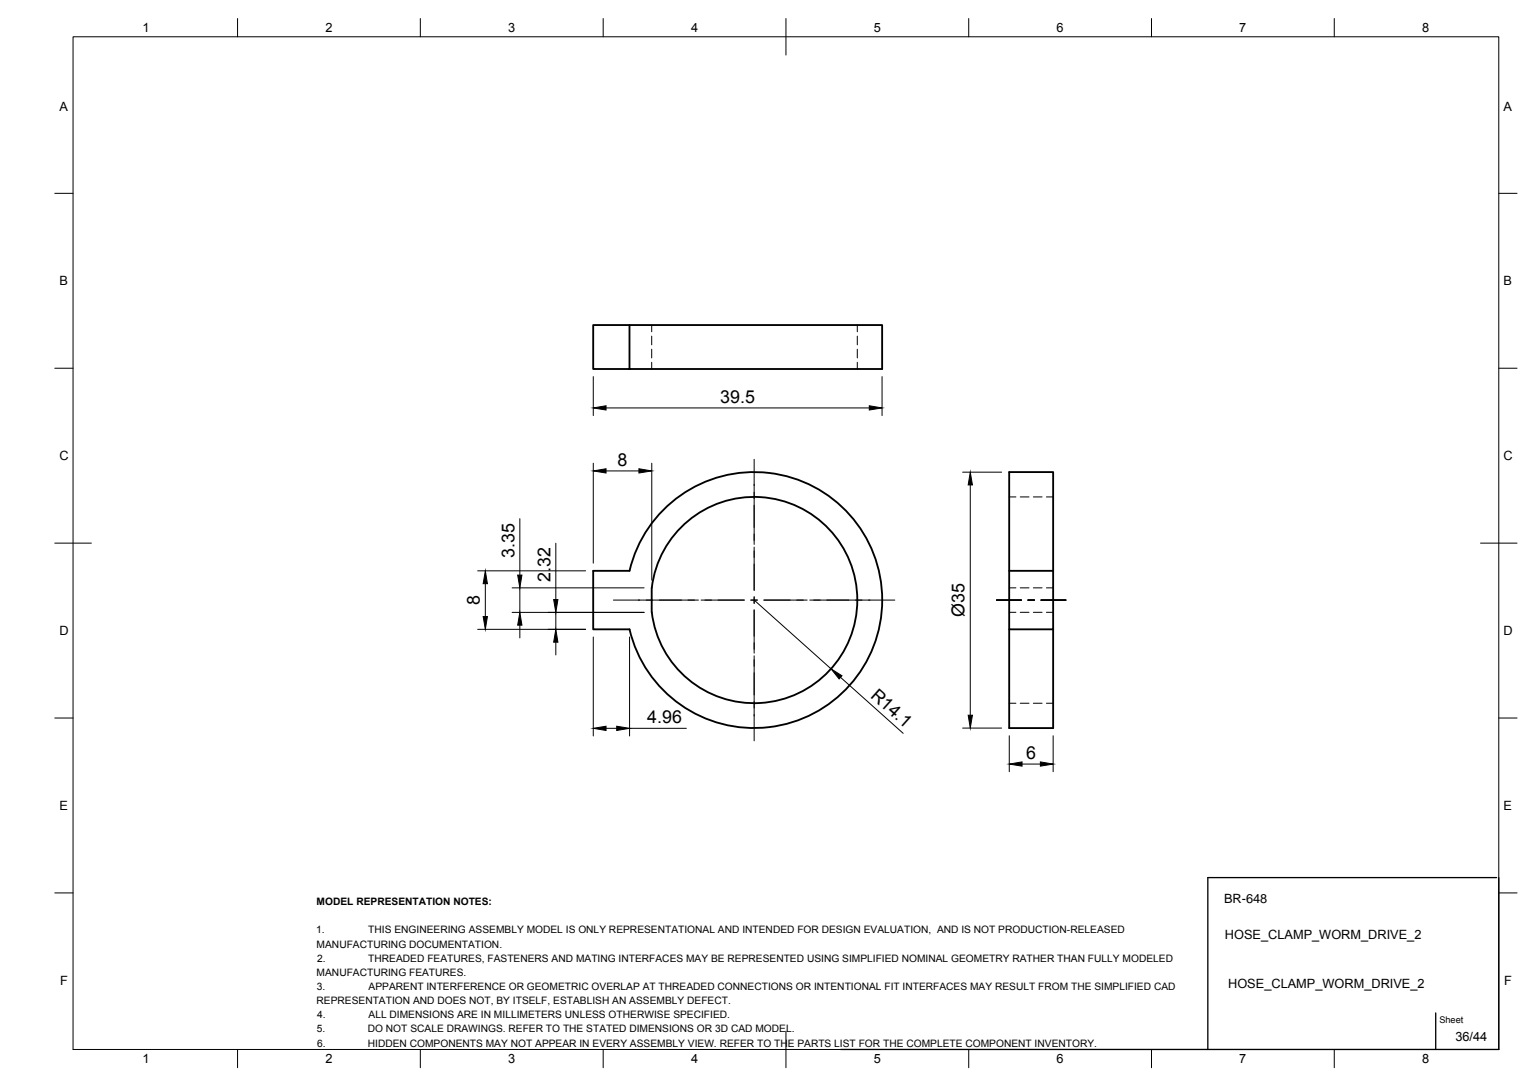
ISO-10303-21;
HEADER;
FILE_DESCRIPTION((''),'2;1');
FILE_NAME('HOSE_CLAMP_WORM_DRIVE_2.step','2026-10-01T22:05:39-07:00',(''),(''),'','','');
FILE_SCHEMA (('AUTOMOTIVE_DESIGN { 1 0 10303 214 3 1 1 }'));
ENDSEC;
DATA;
#10=MECHANICAL_DESIGN_GEOMETRIC_PRESENTATION_REPRESENTATION('',(#634),#24628);
#550=SHAPE_REPRESENTATION_RELATIONSHIP('SRR','None',#24823,#592) ;
#592=ADVANCED_BREP_SHAPE_REPRESENTATION('',(#673),#24613) ;
#634=STYLED_ITEM('',(#25034),#673) ;
#673=MANIFOLD_SOLID_BREP('HOSE_CLAMP_WORM_DRIVE_2',#13176) ;
#906=FACE_BOUND('',#4608,.T.) ;
#907=FACE_BOUND('',#4610,.T.) ;
#1693=LINE('',#23744,#2529) ;
#1694=LINE('',#23746,#2530) ;
#1695=LINE('',#23748,#2531) ;
#1696=LINE('',#23749,#2532) ;
#1697=LINE('',#23753,#2533) ;
#1698=LINE('',#23755,#2534) ;
#1699=LINE('',#23757,#2535) ;
#1700=LINE('',#23758,#2536) ;
#1701=LINE('',#23762,#2537) ;
#1702=LINE('',#23764,#2538) ;
#1703=LINE('',#23766,#2539) ;
#1704=LINE('',#23767,#2540) ;
#1705=LINE('',#23769,#2541) ;
#1706=LINE('',#23770,#2542) ;
#2529=VECTOR('',#19094,1.) ;
#2530=VECTOR('',#19095,1.) ;
#2531=VECTOR('',#19096,1.) ;
#2532=VECTOR('',#19097,1.) ;
#2533=VECTOR('',#19100,1.) ;
#2534=VECTOR('',#19101,1.) ;
#2535=VECTOR('',#19102,1.) ;
#2536=VECTOR('',#19103,1.) ;
#2537=VECTOR('',#19106,1.) ;
#2538=VECTOR('',#19107,1.) ;
#2539=VECTOR('',#19108,1.) ;
#2540=VECTOR('',#19109,1.) ;
#2541=VECTOR('',#19112,1.) ;
#2542=VECTOR('',#19113,1.) ;
#2915=CYLINDRICAL_SURFACE('',#15161,1.75) ;
#2916=CYLINDRICAL_SURFACE('',#15164,1.41) ;
#3614=FACE_OUTER_BOUND('',#4601,.T.) ;
#3615=FACE_OUTER_BOUND('',#4602,.T.) ;
#3616=FACE_OUTER_BOUND('',#4603,.T.) ;
#3617=FACE_OUTER_BOUND('',#4604,.T.) ;
#3618=FACE_OUTER_BOUND('',#4605,.T.) ;
#3619=FACE_OUTER_BOUND('',#4606,.T.) ;
#3620=FACE_OUTER_BOUND('',#4607,.T.) ;
#3621=FACE_OUTER_BOUND('',#4609,.T.) ;
#4601=EDGE_LOOP('',(#11531,#11532,#11533,#11534)) ;
#4602=EDGE_LOOP('',(#11535,#11536,#11537,#11538)) ;
#4603=EDGE_LOOP('',(#11539,#11540,#11541,#11542)) ;
#4604=EDGE_LOOP('',(#11543,#11544,#11545,#11546)) ;
#4605=EDGE_LOOP('',(#11547,#11548,#11549,#11550)) ;
#4606=EDGE_LOOP('',(#11551,#11552,#11553,#11554)) ;
#4607=EDGE_LOOP('',(#11555,#11556,#11557,#11558)) ;
#4608=EDGE_LOOP('',(#11559,#11560)) ;
#4609=EDGE_LOOP('',(#11561,#11562,#11563,#11564)) ;
#4610=EDGE_LOOP('',(#11565,#11566)) ;
#5465=CIRCLE('',#15162,1.75) ;
#5466=CIRCLE('',#15163,1.75) ;
#5467=CIRCLE('',#15165,1.41) ;
#5468=CIRCLE('',#15166,1.41) ;
#6579=VERTEX_POINT('',#23742) ;
#6580=VERTEX_POINT('',#23743) ;
#6581=VERTEX_POINT('',#23745) ;
#6582=VERTEX_POINT('',#23747) ;
#6583=VERTEX_POINT('',#23751) ;
#6584=VERTEX_POINT('',#23752) ;
#6585=VERTEX_POINT('',#23754) ;
#6586=VERTEX_POINT('',#23756) ;
#6587=VERTEX_POINT('',#23760) ;
#6588=VERTEX_POINT('',#23761) ;
#6589=VERTEX_POINT('',#23763) ;
#6590=VERTEX_POINT('',#23765) ;
#8255=EDGE_CURVE('',#6579,#6580,#1693,.T.) ;
#8256=EDGE_CURVE('',#6579,#6581,#1694,.T.) ;
#8257=EDGE_CURVE('',#6581,#6582,#1695,.T.) ;
#8258=EDGE_CURVE('',#6582,#6580,#1696,.T.) ;
#8259=EDGE_CURVE('',#6583,#6584,#1697,.T.) ;
#8260=EDGE_CURVE('',#6585,#6583,#1698,.T.) ;
#8261=EDGE_CURVE('',#6586,#6585,#1699,.T.) ;
#8262=EDGE_CURVE('',#6586,#6584,#1700,.T.) ;
#8263=EDGE_CURVE('',#6587,#6588,#1701,.T.) ;
#8264=EDGE_CURVE('',#6587,#6589,#1702,.T.) ;
#8265=EDGE_CURVE('',#6589,#6590,#1703,.T.) ;
#8266=EDGE_CURVE('',#6590,#6588,#1704,.T.) ;
#8267=EDGE_CURVE('',#6581,#6590,#1705,.T.) ;
#8268=EDGE_CURVE('',#6582,#6589,#1706,.T.) ;
#8269=EDGE_CURVE('',#6579,#6588,#5465,.T.) ;
#8270=EDGE_CURVE('',#6587,#6580,#5466,.T.) ;
#8271=EDGE_CURVE('',#6586,#6584,#5467,.T.) ;
#8272=EDGE_CURVE('',#6583,#6585,#5468,.T.) ;
#11531=ORIENTED_EDGE('',*,*,#8255,.F.) ;
#11532=ORIENTED_EDGE('',*,*,#8256,.T.) ;
#11533=ORIENTED_EDGE('',*,*,#8257,.T.) ;
#11534=ORIENTED_EDGE('',*,*,#8258,.T.) ;
#11535=ORIENTED_EDGE('',*,*,#8259,.F.) ;
#11536=ORIENTED_EDGE('',*,*,#8260,.F.) ;
#11537=ORIENTED_EDGE('',*,*,#8261,.F.) ;
#11538=ORIENTED_EDGE('',*,*,#8262,.T.) ;
#11539=ORIENTED_EDGE('',*,*,#8263,.F.) ;
#11540=ORIENTED_EDGE('',*,*,#8264,.T.) ;
#11541=ORIENTED_EDGE('',*,*,#8265,.T.) ;
#11542=ORIENTED_EDGE('',*,*,#8266,.T.) ;
#11543=ORIENTED_EDGE('',*,*,#8267,.T.) ;
#11544=ORIENTED_EDGE('',*,*,#8265,.F.) ;
#11545=ORIENTED_EDGE('',*,*,#8268,.F.) ;
#11546=ORIENTED_EDGE('',*,*,#8257,.F.) ;
#11547=ORIENTED_EDGE('',*,*,#8263,.T.) ;
#11548=ORIENTED_EDGE('',*,*,#8269,.F.) ;
#11549=ORIENTED_EDGE('',*,*,#8255,.T.) ;
#11550=ORIENTED_EDGE('',*,*,#8270,.F.) ;
#11551=ORIENTED_EDGE('',*,*,#8259,.T.) ;
#11552=ORIENTED_EDGE('',*,*,#8271,.F.) ;
#11553=ORIENTED_EDGE('',*,*,#8261,.T.) ;
#11554=ORIENTED_EDGE('',*,*,#8272,.F.) ;
#11555=ORIENTED_EDGE('',*,*,#8269,.T.) ;
#11556=ORIENTED_EDGE('',*,*,#8266,.F.) ;
#11557=ORIENTED_EDGE('',*,*,#8267,.F.) ;
#11558=ORIENTED_EDGE('',*,*,#8256,.F.) ;
#11559=ORIENTED_EDGE('',*,*,#8272,.T.) ;
#11560=ORIENTED_EDGE('',*,*,#8260,.T.) ;
#11561=ORIENTED_EDGE('',*,*,#8270,.T.) ;
#11562=ORIENTED_EDGE('',*,*,#8258,.F.) ;
#11563=ORIENTED_EDGE('',*,*,#8268,.T.) ;
#11564=ORIENTED_EDGE('',*,*,#8264,.F.) ;
#11565=ORIENTED_EDGE('',*,*,#8271,.T.) ;
#11566=ORIENTED_EDGE('',*,*,#8262,.F.) ;
#12281=PLANE('',#15157) ;
#12282=PLANE('',#15158) ;
#12283=PLANE('',#15159) ;
#12284=PLANE('',#15160) ;
#12285=PLANE('',#15167) ;
#12286=PLANE('',#15168) ;
#13009=ADVANCED_FACE('',(#3614),#12281,.T.) ;
#13010=ADVANCED_FACE('',(#3615),#12282,.F.) ;
#13011=ADVANCED_FACE('',(#3616),#12283,.F.) ;
#13012=ADVANCED_FACE('',(#3617),#12284,.F.) ;
#13013=ADVANCED_FACE('',(#3618),#2915,.T.) ;
#13014=ADVANCED_FACE('',(#3619),#2916,.F.) ;
#13015=ADVANCED_FACE('',(#3620,#906),#12285,.T.) ;
#13016=ADVANCED_FACE('',(#3621,#907),#12286,.T.) ;
#13176=CLOSED_SHELL('',(#13009,#13010,#13011,#13012,#13013,#13014,#13015,
#13016)) ;
#15156=AXIS2_PLACEMENT_3D('',#23740,#19090,#19091) ;
#15157=AXIS2_PLACEMENT_3D('',#23741,#19092,#19093) ;
#15158=AXIS2_PLACEMENT_3D('',#23750,#19098,#19099) ;
#15159=AXIS2_PLACEMENT_3D('',#23759,#19104,#19105) ;
#15160=AXIS2_PLACEMENT_3D('',#23768,#19110,#19111) ;
#15161=AXIS2_PLACEMENT_3D('',#23771,#19114,#19115) ;
#15162=AXIS2_PLACEMENT_3D('',#23772,#19116,#19117) ;
#15163=AXIS2_PLACEMENT_3D('',#23773,#19118,#19119) ;
#15164=AXIS2_PLACEMENT_3D('',#23774,#19120,#19121) ;
#15165=AXIS2_PLACEMENT_3D('',#23775,#19122,#19123) ;
#15166=AXIS2_PLACEMENT_3D('',#23776,#19124,#19125) ;
#15167=AXIS2_PLACEMENT_3D('',#23777,#19126,#19127) ;
#15168=AXIS2_PLACEMENT_3D('',#23778,#19128,#19129) ;
#19090=DIRECTION('axis',(0.,0.,1.)) ;
#19091=DIRECTION('refdir',(1.,0.,0.)) ;
#19092=DIRECTION('center_axis',(0.,0.,1.)) ;
#19093=DIRECTION('ref_axis',(1.,0.,0.)) ;
#19094=DIRECTION('',(0.,1.,0.)) ;
#19095=DIRECTION('',(1.,0.,0.)) ;
#19096=DIRECTION('',(0.,1.,0.)) ;
#19097=DIRECTION('',(-1.,0.,0.)) ;
#19098=DIRECTION('center_axis',(1.,0.,0.)) ;
#19099=DIRECTION('ref_axis',(0.,0.,-1.)) ;
#19100=DIRECTION('',(0.,1.,0.)) ;
#19101=DIRECTION('',(0.,0.,-1.)) ;
#19102=DIRECTION('',(0.,-1.,0.)) ;
#19103=DIRECTION('',(0.,0.,-1.)) ;
#19104=DIRECTION('center_axis',(0.,0.,1.)) ;
#19105=DIRECTION('ref_axis',(1.,0.,0.)) ;
#19106=DIRECTION('',(0.,-1.,0.)) ;
#19107=DIRECTION('',(1.,0.,0.)) ;
#19108=DIRECTION('',(0.,-1.,0.)) ;
#19109=DIRECTION('',(-1.,0.,0.)) ;
#19110=DIRECTION('center_axis',(-1.,0.,0.)) ;
#19111=DIRECTION('ref_axis',(0.,0.,1.)) ;
#19112=DIRECTION('',(0.,0.,-1.)) ;
#19113=DIRECTION('',(0.,0.,-1.)) ;
#19114=DIRECTION('center_axis',(0.,1.,0.)) ;
#19115=DIRECTION('ref_axis',(-1.,0.,-1.22464679914735E-16)) ;
#19116=DIRECTION('center_axis',(0.,-1.,0.)) ;
#19117=DIRECTION('ref_axis',(1.,0.,0.)) ;
#19118=DIRECTION('center_axis',(0.,1.,0.)) ;
#19119=DIRECTION('ref_axis',(1.,0.,0.)) ;
#19120=DIRECTION('center_axis',(0.,1.,0.)) ;
#19121=DIRECTION('ref_axis',(-1.,0.,-5.66553889764798E-16)) ;
#19122=DIRECTION('center_axis',(0.,-1.,0.)) ;
#19123=DIRECTION('ref_axis',(1.,0.,0.)) ;
#19124=DIRECTION('center_axis',(0.,1.,0.)) ;
#19125=DIRECTION('ref_axis',(1.,0.,0.)) ;
#19126=DIRECTION('center_axis',(0.,-1.,0.)) ;
#19127=DIRECTION('ref_axis',(-1.,0.,0.)) ;
#19128=DIRECTION('center_axis',(0.,1.,0.)) ;
#19129=DIRECTION('ref_axis',(1.,0.,0.)) ;
#23740=CARTESIAN_POINT('',(0.,0.,0.)) ;
#23741=CARTESIAN_POINT('Origin',(9.8,-5.4,-7.6)) ;
#23742=CARTESIAN_POINT('',(9.70367250374008,-5.7,-7.6)) ;
#23743=CARTESIAN_POINT('',(9.70367250374008,-5.1,-7.6)) ;
#23744=CARTESIAN_POINT('',(9.70367250374008,-5.4,-7.6)) ;
#23745=CARTESIAN_POINT('',(10.2,-5.7,-7.6)) ;
#23746=CARTESIAN_POINT('',(9.8,-5.7,-7.6)) ;
#23747=CARTESIAN_POINT('',(10.2,-5.1,-7.6)) ;
#23748=CARTESIAN_POINT('',(10.2,-5.4,-7.6)) ;
#23749=CARTESIAN_POINT('',(9.8,-5.1,-7.6)) ;
#23750=CARTESIAN_POINT('Origin',(9.4,-5.4,-8.)) ;
#23751=CARTESIAN_POINT('',(9.4,-5.7,-8.1676305461424)) ;
#23752=CARTESIAN_POINT('',(9.4,-5.1,-8.1676305461424)) ;
#23753=CARTESIAN_POINT('',(9.4,-5.4,-8.1676305461424)) ;
#23754=CARTESIAN_POINT('',(9.4,-5.7,-7.8323694538576)) ;
#23755=CARTESIAN_POINT('',(9.4,-5.7,-8.)) ;
#23756=CARTESIAN_POINT('',(9.4,-5.1,-7.8323694538576)) ;
#23757=CARTESIAN_POINT('',(9.4,-5.4,-7.8323694538576)) ;
#23758=CARTESIAN_POINT('',(9.4,-5.1,-8.)) ;
#23759=CARTESIAN_POINT('Origin',(9.8,-5.4,-8.4)) ;
#23760=CARTESIAN_POINT('',(9.70367250374008,-5.1,-8.4)) ;
#23761=CARTESIAN_POINT('',(9.70367250374008,-5.7,-8.4)) ;
#23762=CARTESIAN_POINT('',(9.70367250374008,-5.4,-8.4)) ;
#23763=CARTESIAN_POINT('',(10.2,-5.1,-8.4)) ;
#23764=CARTESIAN_POINT('',(9.8,-5.1,-8.4)) ;
#23765=CARTESIAN_POINT('',(10.2,-5.7,-8.4)) ;
#23766=CARTESIAN_POINT('',(10.2,-5.4,-8.4)) ;
#23767=CARTESIAN_POINT('',(9.8,-5.7,-8.4)) ;
#23768=CARTESIAN_POINT('Origin',(10.2,-5.4,-8.)) ;
#23769=CARTESIAN_POINT('',(10.2,-5.7,-8.)) ;
#23770=CARTESIAN_POINT('',(10.2,-5.1,-8.)) ;
#23771=CARTESIAN_POINT('Origin',(8.,-5.4,-8.)) ;
#23772=CARTESIAN_POINT('Origin',(8.,-5.7,-8.)) ;
#23773=CARTESIAN_POINT('Origin',(8.,-5.1,-8.)) ;
#23774=CARTESIAN_POINT('Origin',(8.,-5.4,-8.)) ;
#23775=CARTESIAN_POINT('Origin',(8.,-5.1,-8.)) ;
#23776=CARTESIAN_POINT('Origin',(8.,-5.7,-8.)) ;
#23777=CARTESIAN_POINT('Origin',(8.,-5.7,-8.)) ;
#23778=CARTESIAN_POINT('Origin',(8.,-5.1,-8.)) ;
#24565=UNCERTAINTY_MEASURE_WITH_UNIT(LENGTH_MEASURE(0.001),#24629,
'DISTANCE_ACCURACY_VALUE',
'Maximum model space distance between geometric entities at asserted c
onnectivities') ;
#24580=UNCERTAINTY_MEASURE_WITH_UNIT(LENGTH_MEASURE(0.001),#24629,
'DISTANCE_ACCURACY_VALUE',
'Maximum model space distance between geometric entities at asserted c
onnectivities') ;
#24613=(
GEOMETRIC_REPRESENTATION_CONTEXT(3)
GLOBAL_UNCERTAINTY_ASSIGNED_CONTEXT((#24565))
GLOBAL_UNIT_ASSIGNED_CONTEXT((#24629,#24631,#24632))
REPRESENTATION_CONTEXT('','3D')
) ;
#24628=(
GEOMETRIC_REPRESENTATION_CONTEXT(3)
GLOBAL_UNCERTAINTY_ASSIGNED_CONTEXT((#24580))
GLOBAL_UNIT_ASSIGNED_CONTEXT((#24629,#24631,#24632))
REPRESENTATION_CONTEXT('','3D')
) ;
#24629=(
LENGTH_UNIT()
NAMED_UNIT(*)
SI_UNIT(.CENTI.,.METRE.)
) ;
#24631=(
NAMED_UNIT(*)
PLANE_ANGLE_UNIT()
SI_UNIT($,.RADIAN.)
) ;
#24632=(
NAMED_UNIT(*)
SI_UNIT($,.STERADIAN.)
SOLID_ANGLE_UNIT()
) ;
#24665=SHAPE_DEFINITION_REPRESENTATION(#24734,#24823) ;
#24734=PRODUCT_DEFINITION_SHAPE('',$,#24871) ;
#24823=SHAPE_REPRESENTATION('',(#15156),#24613) ;
#24838=PRODUCT_DEFINITION_CONTEXT('part definition',#24981,'design') ;
#24871=PRODUCT_DEFINITION('HOSE_CLAMP_WORM_DRIVE_2',
'HOSE_CLAMP_WORM_DRIVE_2',#24918,#24838) ;
#24918=PRODUCT_DEFINITION_FORMATION('',$,#25015) ;
#24981=APPLICATION_CONTEXT(
'Core Data for Automotive Mechanical Design Process') ;
#24982=PRODUCT_CONTEXT('part definition',#24981,'mechanical') ;
#25015=PRODUCT('HOSE_CLAMP_WORM_DRIVE_2','HOSE_CLAMP_WORM_DRIVE_2',$,(#24982)) ;
#25034=PRESENTATION_STYLE_ASSIGNMENT((#25044)) ;
#25044=SURFACE_STYLE_USAGE(.BOTH.,#25054) ;
#25054=SURFACE_SIDE_STYLE('',(#25064)) ;
#25064=SURFACE_STYLE_FILL_AREA(#25074) ;
#25074=FILL_AREA_STYLE('Stainless Steel - Satin',(#25084)) ;
#25084=FILL_AREA_STYLE_COLOUR('Stainless Steel - Satin',#25094) ;
#25094=COLOUR_RGB('Stainless Steel - Satin', 0.31764706, 0.68627451, 0.89019608) ;
ENDSEC;
END-ISO-10303-21;
